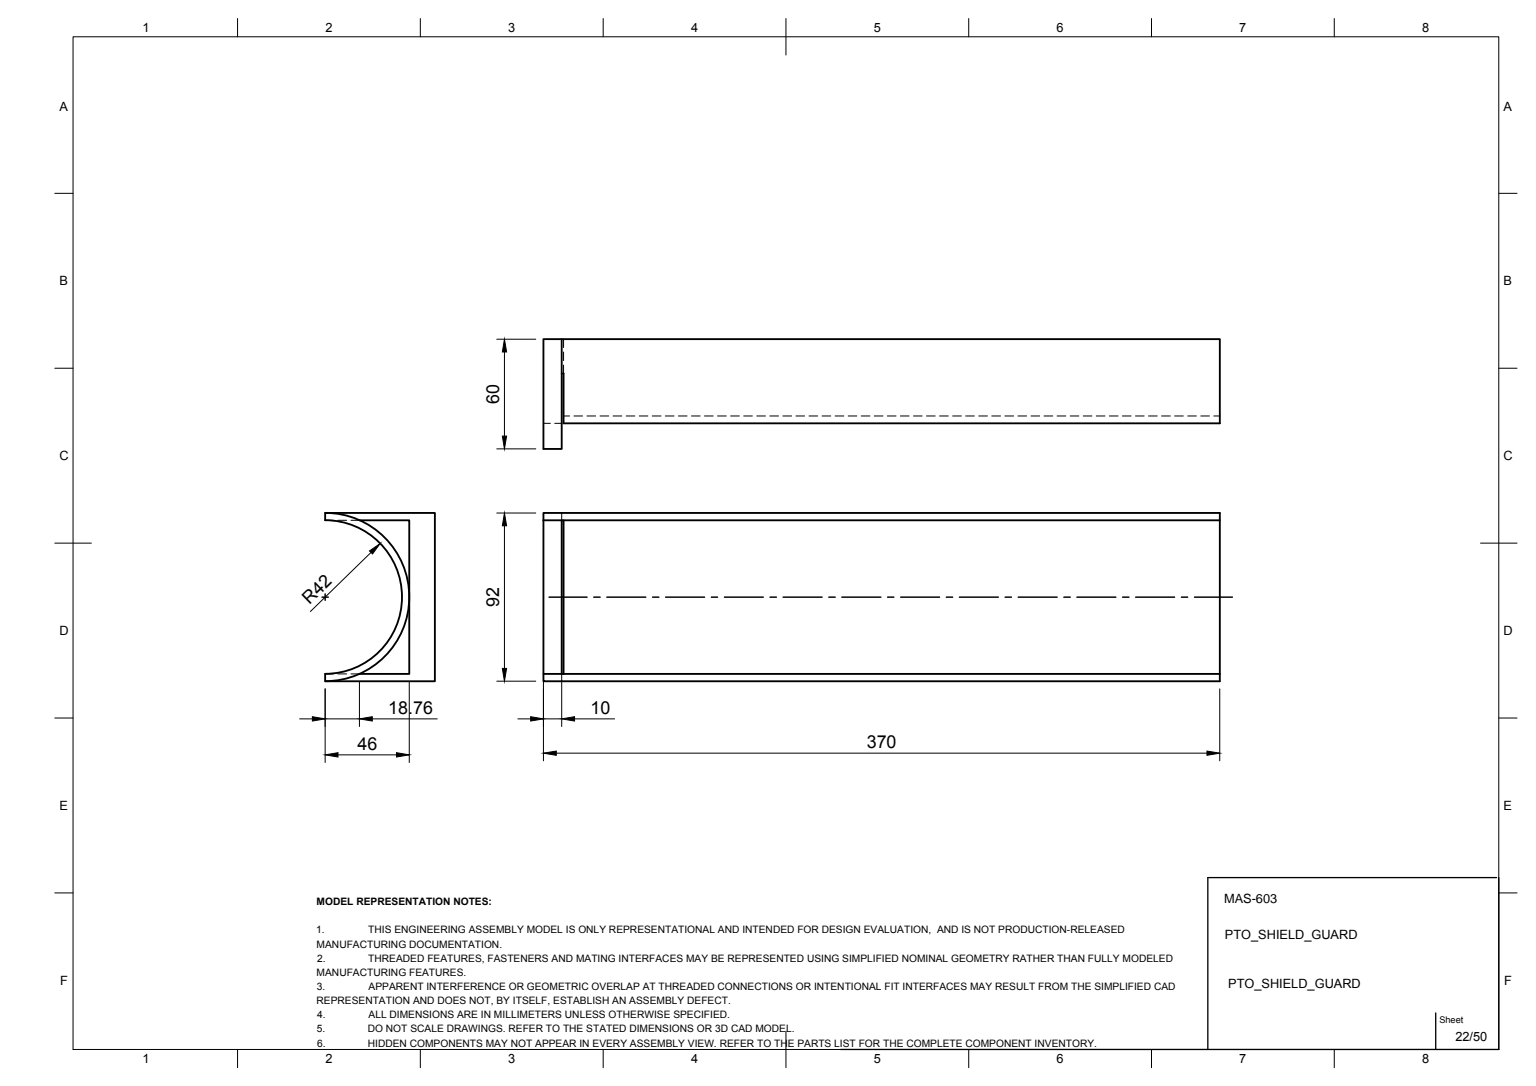
ISO-10303-21;
HEADER;
FILE_DESCRIPTION((''),'2;1');
FILE_NAME('PTO_SHIELD_GUARD.step','2026-10-01T22:06:14-07:00',(''),(''),'','','');
FILE_SCHEMA (('AUTOMOTIVE_DESIGN { 1 0 10303 214 3 1 1 }'));
ENDSEC;
DATA;
#10=MECHANICAL_DESIGN_GEOMETRIC_PRESENTATION_REPRESENTATION('',(#994),#50440);
#904=SHAPE_REPRESENTATION_RELATIONSHIP('SRR','None',#50636,#949) ;
#949=ADVANCED_BREP_SHAPE_REPRESENTATION('',(#1049),#50405) ;
#994=STYLED_ITEM('',(#50884),#1049) ;
#1049=MANIFOLD_SOLID_BREP('PTO_SHIELD_GUARD',#28661) ;
#2034=PLANE('',#30519) ;
#2035=PLANE('',#30522) ;
#2036=PLANE('',#30523) ;
#2037=PLANE('',#30524) ;
#2038=PLANE('',#30531) ;
#2039=PLANE('',#30532) ;
#2040=PLANE('',#30533) ;
#2041=PLANE('',#30534) ;
#2042=PLANE('',#30535) ;
#2043=PLANE('',#30536) ;
#2044=PLANE('',#30537) ;
#2045=PLANE('',#30538) ;
#3164=FACE_OUTER_BOUND('',#4905,.T.) ;
#3165=FACE_OUTER_BOUND('',#4906,.T.) ;
#3166=FACE_OUTER_BOUND('',#4907,.T.) ;
#3167=FACE_OUTER_BOUND('',#4908,.T.) ;
#3168=FACE_OUTER_BOUND('',#4909,.T.) ;
#3169=FACE_OUTER_BOUND('',#4910,.T.) ;
#3170=FACE_OUTER_BOUND('',#4911,.T.) ;
#3171=FACE_OUTER_BOUND('',#4912,.T.) ;
#3172=FACE_OUTER_BOUND('',#4913,.T.) ;
#3173=FACE_OUTER_BOUND('',#4914,.T.) ;
#3174=FACE_OUTER_BOUND('',#4915,.T.) ;
#3175=FACE_OUTER_BOUND('',#4916,.T.) ;
#3176=FACE_OUTER_BOUND('',#4917,.T.) ;
#3177=FACE_OUTER_BOUND('',#4918,.T.) ;
#4905=EDGE_LOOP('',(#22873,#22874,#22875,#22876)) ;
#4906=EDGE_LOOP('',(#22877,#22878,#22879,#22880,#22881,#22882)) ;
#4907=EDGE_LOOP('',(#22883,#22884,#22885,#22886)) ;
#4908=EDGE_LOOP('',(#22887,#22888,#22889,#22890,#22891,#22892)) ;
#4909=EDGE_LOOP('',(#22893,#22894,#22895,#22896,#22897,#22898,#22899,#22900)) ;
#4910=EDGE_LOOP('',(#22901,#22902,#22903,#22904)) ;
#4911=EDGE_LOOP('',(#22905,#22906,#22907,#22908,#22909,#22910)) ;
#4912=EDGE_LOOP('',(#22911,#22912,#22913,#22914,#22915,#22916,#22917,#22918)) ;
#4913=EDGE_LOOP('',(#22919,#22920,#22921,#22922,#22923,#22924,#22925,#22926)) ;
#4914=EDGE_LOOP('',(#22927,#22928,#22929,#22930)) ;
#4915=EDGE_LOOP('',(#22931,#22932,#22933,#22934)) ;
#4916=EDGE_LOOP('',(#22935,#22936,#22937,#22938)) ;
#4917=EDGE_LOOP('',(#22939,#22940,#22941,#22942,#22943,#22944)) ;
#4918=EDGE_LOOP('',(#22945,#22946,#22947,#22948)) ;
#7409=LINE('',#45813,#9881) ;
#7410=LINE('',#45816,#9882) ;
#7411=LINE('',#45819,#9883) ;
#7412=LINE('',#45821,#9884) ;
#7413=LINE('',#45823,#9885) ;
#7414=LINE('',#45825,#9886) ;
#7415=LINE('',#45826,#9887) ;
#7416=LINE('',#45829,#9888) ;
#7417=LINE('',#45831,#9889) ;
#7418=LINE('',#45832,#9890) ;
#7419=LINE('',#45835,#9891) ;
#7420=LINE('',#45836,#9892) ;
#7421=LINE('',#45838,#9893) ;
#7422=LINE('',#45839,#9894) ;
#7423=LINE('',#45844,#9895) ;
#7424=LINE('',#45848,#9896) ;
#7425=LINE('',#45852,#9897) ;
#7426=LINE('',#45855,#9898) ;
#7427=LINE('',#45858,#9899) ;
#7428=LINE('',#45859,#9900) ;
#7429=LINE('',#45860,#9901) ;
#7430=LINE('',#45863,#9902) ;
#7431=LINE('',#45865,#9903) ;
#7432=LINE('',#45867,#9904) ;
#7433=LINE('',#45868,#9905) ;
#7434=LINE('',#45871,#9906) ;
#7435=LINE('',#45873,#9907) ;
#7436=LINE('',#45874,#9908) ;
#7437=LINE('',#45876,#9909) ;
#7438=LINE('',#45877,#9910) ;
#7439=LINE('',#45880,#9911) ;
#7440=LINE('',#45882,#9912) ;
#9881=VECTOR('',#36676,1.) ;
#9882=VECTOR('',#36679,1.) ;
#9883=VECTOR('',#36682,1.) ;
#9884=VECTOR('',#36683,1.) ;
#9885=VECTOR('',#36684,1.) ;
#9886=VECTOR('',#36685,1.) ;
#9887=VECTOR('',#36686,1.) ;
#9888=VECTOR('',#36689,1.) ;
#9889=VECTOR('',#36690,1.) ;
#9890=VECTOR('',#36691,1.) ;
#9891=VECTOR('',#36694,1.) ;
#9892=VECTOR('',#36695,1.) ;
#9893=VECTOR('',#36696,1.) ;
#9894=VECTOR('',#36697,1.) ;
#9895=VECTOR('',#36702,1.) ;
#9896=VECTOR('',#36705,1.) ;
#9897=VECTOR('',#36710,1.) ;
#9898=VECTOR('',#36713,1.) ;
#9899=VECTOR('',#36716,1.) ;
#9900=VECTOR('',#36717,1.) ;
#9901=VECTOR('',#36718,1.) ;
#9902=VECTOR('',#36721,1.) ;
#9903=VECTOR('',#36722,1.) ;
#9904=VECTOR('',#36723,1.) ;
#9905=VECTOR('',#36724,1.) ;
#9906=VECTOR('',#36727,1.) ;
#9907=VECTOR('',#36728,1.) ;
#9908=VECTOR('',#36729,1.) ;
#9909=VECTOR('',#36732,1.) ;
#9910=VECTOR('',#36733,1.) ;
#9911=VECTOR('',#36738,1.) ;
#9912=VECTOR('',#36741,1.) ;
#11097=CIRCLE('',#30520,4.6) ;
#11098=CIRCLE('',#30521,4.2) ;
#11099=CIRCLE('',#30526,4.6) ;
#11100=CIRCLE('',#30527,4.6) ;
#11101=CIRCLE('',#30528,4.6) ;
#11102=CIRCLE('',#30530,4.2) ;
#13275=VERTEX_POINT('',#45809) ;
#13276=VERTEX_POINT('',#45810) ;
#13277=VERTEX_POINT('',#45812) ;
#13278=VERTEX_POINT('',#45814) ;
#13279=VERTEX_POINT('',#45818) ;
#13280=VERTEX_POINT('',#45820) ;
#13281=VERTEX_POINT('',#45822) ;
#13282=VERTEX_POINT('',#45824) ;
#13283=VERTEX_POINT('',#45828) ;
#13284=VERTEX_POINT('',#45830) ;
#13285=VERTEX_POINT('',#45834) ;
#13286=VERTEX_POINT('',#45837) ;
#13287=VERTEX_POINT('',#45841) ;
#13288=VERTEX_POINT('',#45843) ;
#13289=VERTEX_POINT('',#45845) ;
#13290=VERTEX_POINT('',#45847) ;
#13291=VERTEX_POINT('',#45851) ;
#13292=VERTEX_POINT('',#45853) ;
#13293=VERTEX_POINT('',#45857) ;
#13294=VERTEX_POINT('',#45862) ;
#13295=VERTEX_POINT('',#45864) ;
#13296=VERTEX_POINT('',#45866) ;
#13297=VERTEX_POINT('',#45870) ;
#13298=VERTEX_POINT('',#45872) ;
#16702=EDGE_CURVE('',#13275,#13276,#11097,.T.) ;
#16703=EDGE_CURVE('',#13275,#13277,#7409,.T.) ;
#16704=EDGE_CURVE('',#13278,#13277,#11098,.T.) ;
#16705=EDGE_CURVE('',#13276,#13278,#7410,.T.) ;
#16706=EDGE_CURVE('',#13276,#13279,#7411,.T.) ;
#16707=EDGE_CURVE('',#13278,#13280,#7412,.T.) ;
#16708=EDGE_CURVE('',#13281,#13280,#7413,.T.) ;
#16709=EDGE_CURVE('',#13281,#13282,#7414,.T.) ;
#16710=EDGE_CURVE('',#13279,#13282,#7415,.T.) ;
#16711=EDGE_CURVE('',#13282,#13283,#7416,.T.) ;
#16712=EDGE_CURVE('',#13284,#13281,#7417,.T.) ;
#16713=EDGE_CURVE('',#13283,#13284,#7418,.T.) ;
#16714=EDGE_CURVE('',#13285,#13275,#7419,.T.) ;
#16715=EDGE_CURVE('',#13283,#13285,#7420,.T.) ;
#16716=EDGE_CURVE('',#13286,#13284,#7421,.T.) ;
#16717=EDGE_CURVE('',#13286,#13277,#7422,.T.) ;
#16718=EDGE_CURVE('',#13279,#13287,#11099,.T.) ;
#16719=EDGE_CURVE('',#13287,#13288,#7423,.T.) ;
#16720=EDGE_CURVE('',#13289,#13288,#11100,.T.) ;
#16721=EDGE_CURVE('',#13289,#13290,#7424,.T.) ;
#16722=EDGE_CURVE('',#13290,#13285,#11101,.T.) ;
#16723=EDGE_CURVE('',#13277,#13291,#7425,.T.) ;
#16724=EDGE_CURVE('',#13292,#13291,#11102,.T.) ;
#16725=EDGE_CURVE('',#13292,#13278,#7426,.T.) ;
#16726=EDGE_CURVE('',#13293,#13286,#7427,.T.) ;
#16727=EDGE_CURVE('',#13290,#13293,#7428,.T.) ;
#16728=EDGE_CURVE('',#13291,#13289,#7429,.T.) ;
#16729=EDGE_CURVE('',#13280,#13294,#7430,.T.) ;
#16730=EDGE_CURVE('',#13295,#13294,#7431,.T.) ;
#16731=EDGE_CURVE('',#13296,#13295,#7432,.T.) ;
#16732=EDGE_CURVE('',#13296,#13293,#7433,.T.) ;
#16733=EDGE_CURVE('',#13297,#13290,#7434,.T.) ;
#16734=EDGE_CURVE('',#13298,#13297,#7435,.T.) ;
#16735=EDGE_CURVE('',#13298,#13287,#7436,.T.) ;
#16736=EDGE_CURVE('',#13295,#13298,#7437,.T.) ;
#16737=EDGE_CURVE('',#13297,#13296,#7438,.T.) ;
#16738=EDGE_CURVE('',#13294,#13287,#7439,.T.) ;
#16739=EDGE_CURVE('',#13288,#13292,#7440,.T.) ;
#22873=ORIENTED_EDGE('',*,*,#16702,.F.) ;
#22874=ORIENTED_EDGE('',*,*,#16703,.T.) ;
#22875=ORIENTED_EDGE('',*,*,#16704,.F.) ;
#22876=ORIENTED_EDGE('',*,*,#16705,.F.) ;
#22877=ORIENTED_EDGE('',*,*,#16706,.F.) ;
#22878=ORIENTED_EDGE('',*,*,#16705,.T.) ;
#22879=ORIENTED_EDGE('',*,*,#16707,.T.) ;
#22880=ORIENTED_EDGE('',*,*,#16708,.F.) ;
#22881=ORIENTED_EDGE('',*,*,#16709,.T.) ;
#22882=ORIENTED_EDGE('',*,*,#16710,.F.) ;
#22883=ORIENTED_EDGE('',*,*,#16711,.F.) ;
#22884=ORIENTED_EDGE('',*,*,#16709,.F.) ;
#22885=ORIENTED_EDGE('',*,*,#16712,.F.) ;
#22886=ORIENTED_EDGE('',*,*,#16713,.F.) ;
#22887=ORIENTED_EDGE('',*,*,#16714,.F.) ;
#22888=ORIENTED_EDGE('',*,*,#16715,.F.) ;
#22889=ORIENTED_EDGE('',*,*,#16713,.T.) ;
#22890=ORIENTED_EDGE('',*,*,#16716,.F.) ;
#22891=ORIENTED_EDGE('',*,*,#16717,.T.) ;
#22892=ORIENTED_EDGE('',*,*,#16703,.F.) ;
#22893=ORIENTED_EDGE('',*,*,#16714,.T.) ;
#22894=ORIENTED_EDGE('',*,*,#16702,.T.) ;
#22895=ORIENTED_EDGE('',*,*,#16706,.T.) ;
#22896=ORIENTED_EDGE('',*,*,#16718,.T.) ;
#22897=ORIENTED_EDGE('',*,*,#16719,.T.) ;
#22898=ORIENTED_EDGE('',*,*,#16720,.F.) ;
#22899=ORIENTED_EDGE('',*,*,#16721,.T.) ;
#22900=ORIENTED_EDGE('',*,*,#16722,.T.) ;
#22901=ORIENTED_EDGE('',*,*,#16704,.T.) ;
#22902=ORIENTED_EDGE('',*,*,#16723,.T.) ;
#22903=ORIENTED_EDGE('',*,*,#16724,.F.) ;
#22904=ORIENTED_EDGE('',*,*,#16725,.T.) ;
#22905=ORIENTED_EDGE('',*,*,#16717,.F.) ;
#22906=ORIENTED_EDGE('',*,*,#16726,.F.) ;
#22907=ORIENTED_EDGE('',*,*,#16727,.F.) ;
#22908=ORIENTED_EDGE('',*,*,#16721,.F.) ;
#22909=ORIENTED_EDGE('',*,*,#16728,.F.) ;
#22910=ORIENTED_EDGE('',*,*,#16723,.F.) ;
#22911=ORIENTED_EDGE('',*,*,#16716,.T.) ;
#22912=ORIENTED_EDGE('',*,*,#16712,.T.) ;
#22913=ORIENTED_EDGE('',*,*,#16708,.T.) ;
#22914=ORIENTED_EDGE('',*,*,#16729,.T.) ;
#22915=ORIENTED_EDGE('',*,*,#16730,.F.) ;
#22916=ORIENTED_EDGE('',*,*,#16731,.F.) ;
#22917=ORIENTED_EDGE('',*,*,#16732,.T.) ;
#22918=ORIENTED_EDGE('',*,*,#16726,.T.) ;
#22919=ORIENTED_EDGE('',*,*,#16715,.T.) ;
#22920=ORIENTED_EDGE('',*,*,#16722,.F.) ;
#22921=ORIENTED_EDGE('',*,*,#16733,.F.) ;
#22922=ORIENTED_EDGE('',*,*,#16734,.F.) ;
#22923=ORIENTED_EDGE('',*,*,#16735,.T.) ;
#22924=ORIENTED_EDGE('',*,*,#16718,.F.) ;
#22925=ORIENTED_EDGE('',*,*,#16710,.T.) ;
#22926=ORIENTED_EDGE('',*,*,#16711,.T.) ;
#22927=ORIENTED_EDGE('',*,*,#16731,.T.) ;
#22928=ORIENTED_EDGE('',*,*,#16736,.T.) ;
#22929=ORIENTED_EDGE('',*,*,#16734,.T.) ;
#22930=ORIENTED_EDGE('',*,*,#16737,.T.) ;
#22931=ORIENTED_EDGE('',*,*,#16733,.T.) ;
#22932=ORIENTED_EDGE('',*,*,#16727,.T.) ;
#22933=ORIENTED_EDGE('',*,*,#16732,.F.) ;
#22934=ORIENTED_EDGE('',*,*,#16737,.F.) ;
#22935=ORIENTED_EDGE('',*,*,#16730,.T.) ;
#22936=ORIENTED_EDGE('',*,*,#16738,.T.) ;
#22937=ORIENTED_EDGE('',*,*,#16735,.F.) ;
#22938=ORIENTED_EDGE('',*,*,#16736,.F.) ;
#22939=ORIENTED_EDGE('',*,*,#16707,.F.) ;
#22940=ORIENTED_EDGE('',*,*,#16725,.F.) ;
#22941=ORIENTED_EDGE('',*,*,#16739,.F.) ;
#22942=ORIENTED_EDGE('',*,*,#16719,.F.) ;
#22943=ORIENTED_EDGE('',*,*,#16738,.F.) ;
#22944=ORIENTED_EDGE('',*,*,#16729,.F.) ;
#22945=ORIENTED_EDGE('',*,*,#16739,.T.) ;
#22946=ORIENTED_EDGE('',*,*,#16724,.T.) ;
#22947=ORIENTED_EDGE('',*,*,#16728,.T.) ;
#22948=ORIENTED_EDGE('',*,*,#16720,.T.) ;
#26819=CYLINDRICAL_SURFACE('',#30525,4.6) ;
#26820=CYLINDRICAL_SURFACE('',#30529,4.2) ;
#27899=ADVANCED_FACE('',(#3164),#2034,.T.) ;
#27900=ADVANCED_FACE('',(#3165),#2035,.T.) ;
#27901=ADVANCED_FACE('',(#3166),#2036,.F.) ;
#27902=ADVANCED_FACE('',(#3167),#2037,.T.) ;
#27903=ADVANCED_FACE('',(#3168),#26819,.T.) ;
#27904=ADVANCED_FACE('',(#3169),#26820,.F.) ;
#27905=ADVANCED_FACE('',(#3170),#2038,.F.) ;
#27906=ADVANCED_FACE('',(#3171),#2039,.T.) ;
#27907=ADVANCED_FACE('',(#3172),#2040,.F.) ;
#27908=ADVANCED_FACE('',(#3173),#2041,.T.) ;
#27909=ADVANCED_FACE('',(#3174),#2042,.F.) ;
#27910=ADVANCED_FACE('',(#3175),#2043,.F.) ;
#27911=ADVANCED_FACE('',(#3176),#2044,.F.) ;
#27912=ADVANCED_FACE('',(#3177),#2045,.T.) ;
#28661=CLOSED_SHELL('',(#27899,#27900,#27901,#27902,#27903,#27904,#27905,
#27906,#27907,#27908,#27909,#27910,#27911,#27912)) ;
#30518=AXIS2_PLACEMENT_3D('',#45807,#36670,#36671) ;
#30519=AXIS2_PLACEMENT_3D('',#45808,#36672,#36673) ;
#30520=AXIS2_PLACEMENT_3D('',#45811,#36674,#36675) ;
#30521=AXIS2_PLACEMENT_3D('',#45815,#36677,#36678) ;
#30522=AXIS2_PLACEMENT_3D('',#45817,#36680,#36681) ;
#30523=AXIS2_PLACEMENT_3D('',#45827,#36687,#36688) ;
#30524=AXIS2_PLACEMENT_3D('',#45833,#36692,#36693) ;
#30525=AXIS2_PLACEMENT_3D('',#45840,#36698,#36699) ;
#30526=AXIS2_PLACEMENT_3D('',#45842,#36700,#36701) ;
#30527=AXIS2_PLACEMENT_3D('',#45846,#36703,#36704) ;
#30528=AXIS2_PLACEMENT_3D('',#45849,#36706,#36707) ;
#30529=AXIS2_PLACEMENT_3D('',#45850,#36708,#36709) ;
#30530=AXIS2_PLACEMENT_3D('',#45854,#36711,#36712) ;
#30531=AXIS2_PLACEMENT_3D('',#45856,#36714,#36715) ;
#30532=AXIS2_PLACEMENT_3D('',#45861,#36719,#36720) ;
#30533=AXIS2_PLACEMENT_3D('',#45869,#36725,#36726) ;
#30534=AXIS2_PLACEMENT_3D('',#45875,#36730,#36731) ;
#30535=AXIS2_PLACEMENT_3D('',#45878,#36734,#36735) ;
#30536=AXIS2_PLACEMENT_3D('',#45879,#36736,#36737) ;
#30537=AXIS2_PLACEMENT_3D('',#45881,#36739,#36740) ;
#30538=AXIS2_PLACEMENT_3D('',#45883,#36742,#36743) ;
#36670=DIRECTION('axis',(0.,0.,1.)) ;
#36671=DIRECTION('refdir',(1.,0.,0.)) ;
#36672=DIRECTION('center_axis',(1.,0.,0.)) ;
#36673=DIRECTION('ref_axis',(0.,0.,-1.)) ;
#36674=DIRECTION('center_axis',(-1.,0.,0.)) ;
#36675=DIRECTION('ref_axis',(0.,0.,-1.)) ;
#36676=DIRECTION('',(0.,0.,-1.)) ;
#36677=DIRECTION('center_axis',(1.,0.,0.)) ;
#36678=DIRECTION('ref_axis',(0.,0.,-1.)) ;
#36679=DIRECTION('',(0.,0.,-1.)) ;
#36680=DIRECTION('center_axis',(0.,-1.,0.)) ;
#36681=DIRECTION('ref_axis',(0.,0.,-1.)) ;
#36682=DIRECTION('',(1.,0.,0.)) ;
#36683=DIRECTION('',(1.,0.,0.)) ;
#36684=DIRECTION('',(0.,0.,-1.)) ;
#36685=DIRECTION('',(-1.,0.,0.)) ;
#36686=DIRECTION('',(0.,0.,1.)) ;
#36687=DIRECTION('center_axis',(0.,0.,1.)) ;
#36688=DIRECTION('ref_axis',(1.,0.,0.)) ;
#36689=DIRECTION('',(0.,-1.,0.)) ;
#36690=DIRECTION('',(0.,1.,0.)) ;
#36691=DIRECTION('',(1.,0.,0.)) ;
#36692=DIRECTION('center_axis',(0.,1.,0.)) ;
#36693=DIRECTION('ref_axis',(0.,0.,1.)) ;
#36694=DIRECTION('',(-1.,0.,0.)) ;
#36695=DIRECTION('',(0.,0.,-1.)) ;
#36696=DIRECTION('',(0.,0.,1.)) ;
#36697=DIRECTION('',(-1.,0.,0.)) ;
#36698=DIRECTION('center_axis',(1.,0.,0.)) ;
#36699=DIRECTION('ref_axis',(0.,-1.22464679914735E-16,1.)) ;
#36700=DIRECTION('center_axis',(-1.,0.,0.)) ;
#36701=DIRECTION('ref_axis',(0.,0.,-1.)) ;
#36702=DIRECTION('',(-1.,0.,0.)) ;
#36703=DIRECTION('center_axis',(-1.,0.,0.)) ;
#36704=DIRECTION('ref_axis',(0.,0.,-1.)) ;
#36705=DIRECTION('',(1.,0.,0.)) ;
#36706=DIRECTION('center_axis',(-1.,0.,0.)) ;
#36707=DIRECTION('ref_axis',(0.,0.,-1.)) ;
#36708=DIRECTION('center_axis',(1.,0.,0.)) ;
#36709=DIRECTION('ref_axis',(0.,1.22464679914735E-16,1.)) ;
#36710=DIRECTION('',(-1.,0.,0.)) ;
#36711=DIRECTION('center_axis',(1.,0.,0.)) ;
#36712=DIRECTION('ref_axis',(0.,0.,-1.)) ;
#36713=DIRECTION('',(1.,0.,0.)) ;
#36714=DIRECTION('center_axis',(0.,0.,1.)) ;
#36715=DIRECTION('ref_axis',(1.,0.,0.)) ;
#36716=DIRECTION('',(0.,1.,0.)) ;
#36717=DIRECTION('',(1.,0.,0.)) ;
#36718=DIRECTION('',(0.,-1.,0.)) ;
#36719=DIRECTION('center_axis',(1.,0.,0.)) ;
#36720=DIRECTION('ref_axis',(0.,0.,-1.)) ;
#36721=DIRECTION('',(0.,1.,0.)) ;
#36722=DIRECTION('',(0.,0.,-1.)) ;
#36723=DIRECTION('',(0.,1.,0.)) ;
#36724=DIRECTION('',(0.,0.,-1.)) ;
#36725=DIRECTION('center_axis',(1.,0.,0.)) ;
#36726=DIRECTION('ref_axis',(0.,0.,-1.)) ;
#36727=DIRECTION('',(0.,0.,-1.)) ;
#36728=DIRECTION('',(0.,-1.,0.)) ;
#36729=DIRECTION('',(0.,0.,-1.)) ;
#36730=DIRECTION('center_axis',(0.,0.,1.)) ;
#36731=DIRECTION('ref_axis',(1.,0.,0.)) ;
#36732=DIRECTION('',(-1.,0.,0.)) ;
#36733=DIRECTION('',(1.,0.,0.)) ;
#36734=DIRECTION('center_axis',(0.,1.,0.)) ;
#36735=DIRECTION('ref_axis',(0.,0.,1.)) ;
#36736=DIRECTION('center_axis',(0.,-1.,0.)) ;
#36737=DIRECTION('ref_axis',(0.,0.,-1.)) ;
#36738=DIRECTION('',(-1.,0.,0.)) ;
#36739=DIRECTION('center_axis',(0.,0.,1.)) ;
#36740=DIRECTION('ref_axis',(1.,0.,0.)) ;
#36741=DIRECTION('',(0.,-1.,0.)) ;
#36742=DIRECTION('center_axis',(-1.,0.,0.)) ;
#36743=DIRECTION('ref_axis',(0.,0.,1.)) ;
#45807=CARTESIAN_POINT('',(0.,0.,0.)) ;
#45808=CARTESIAN_POINT('Origin',(-16.1,0.,36.3)) ;
#45809=CARTESIAN_POINT('',(-16.1,-4.2,35.8761663039294)) ;
#45810=CARTESIAN_POINT('',(-16.1,4.2,35.8761663039294)) ;
#45811=CARTESIAN_POINT('Origin',(-16.1,0.,34.)) ;
#45812=CARTESIAN_POINT('',(-16.1,-4.2,34.)) ;
#45813=CARTESIAN_POINT('',(-16.1,-4.2,36.3)) ;
#45814=CARTESIAN_POINT('',(-16.1,4.2,34.)) ;
#45815=CARTESIAN_POINT('Origin',(-16.1,0.,34.)) ;
#45816=CARTESIAN_POINT('',(-16.1,4.2,36.3)) ;
#45817=CARTESIAN_POINT('Origin',(-15.5,4.2,36.3)) ;
#45818=CARTESIAN_POINT('',(-16.,4.2,35.8761663039294)) ;
#45819=CARTESIAN_POINT('',(-33.5,4.2,35.8761663039294)) ;
#45820=CARTESIAN_POINT('',(-15.,4.2,34.)) ;
#45821=CARTESIAN_POINT('',(-33.5,4.2,34.)) ;
#45822=CARTESIAN_POINT('',(-15.,4.2,38.6)) ;
#45823=CARTESIAN_POINT('',(-15.,4.2,35.15)) ;
#45824=CARTESIAN_POINT('',(-16.,4.2,38.6)) ;
#45825=CARTESIAN_POINT('',(-15.5,4.2,38.6)) ;
#45826=CARTESIAN_POINT('',(-16.,4.2,36.65)) ;
#45827=CARTESIAN_POINT('Origin',(-15.5,0.,38.6)) ;
#45828=CARTESIAN_POINT('',(-16.,-4.2,38.6)) ;
#45829=CARTESIAN_POINT('',(-16.,0.,38.6)) ;
#45830=CARTESIAN_POINT('',(-15.,-4.2,38.6)) ;
#45831=CARTESIAN_POINT('',(-15.,0.,38.6)) ;
#45832=CARTESIAN_POINT('',(-15.5,-4.2,38.6)) ;
#45833=CARTESIAN_POINT('Origin',(-15.5,-4.2,36.3)) ;
#45834=CARTESIAN_POINT('',(-16.,-4.2,35.8761663039294)) ;
#45835=CARTESIAN_POINT('',(-33.5,-4.2,35.8761663039294)) ;
#45836=CARTESIAN_POINT('',(-16.,-4.2,36.65)) ;
#45837=CARTESIAN_POINT('',(-15.,-4.2,34.)) ;
#45838=CARTESIAN_POINT('',(-15.,-4.2,35.15)) ;
#45839=CARTESIAN_POINT('',(-33.5,-4.2,34.)) ;
#45840=CARTESIAN_POINT('Origin',(-33.5,0.,34.)) ;
#45841=CARTESIAN_POINT('',(-16.,4.6,34.)) ;
#45842=CARTESIAN_POINT('Origin',(-16.,0.,34.)) ;
#45843=CARTESIAN_POINT('',(-52.,4.6,34.)) ;
#45844=CARTESIAN_POINT('',(-33.5,4.6,34.)) ;
#45845=CARTESIAN_POINT('',(-52.,-4.6,34.)) ;
#45846=CARTESIAN_POINT('Origin',(-52.,0.,34.)) ;
#45847=CARTESIAN_POINT('',(-16.,-4.6,34.)) ;
#45848=CARTESIAN_POINT('',(-33.5,-4.6,34.)) ;
#45849=CARTESIAN_POINT('Origin',(-16.,0.,34.)) ;
#45850=CARTESIAN_POINT('Origin',(-33.5,0.,34.)) ;
#45851=CARTESIAN_POINT('',(-52.,-4.2,34.)) ;
#45852=CARTESIAN_POINT('',(-33.5,-4.2,34.)) ;
#45853=CARTESIAN_POINT('',(-52.,4.2,34.)) ;
#45854=CARTESIAN_POINT('Origin',(-52.,0.,34.)) ;
#45855=CARTESIAN_POINT('',(-33.5,4.2,34.)) ;
#45856=CARTESIAN_POINT('Origin',(-33.5,0.,34.)) ;
#45857=CARTESIAN_POINT('',(-15.,-4.6,34.)) ;
#45858=CARTESIAN_POINT('',(-15.,0.,34.)) ;
#45859=CARTESIAN_POINT('',(-33.5,-4.6,34.)) ;
#45860=CARTESIAN_POINT('',(-52.,0.,34.)) ;
#45861=CARTESIAN_POINT('Origin',(-15.,0.,34.)) ;
#45862=CARTESIAN_POINT('',(-15.,4.6,34.)) ;
#45863=CARTESIAN_POINT('',(-15.,0.,34.)) ;
#45864=CARTESIAN_POINT('',(-15.,4.6,40.)) ;
#45865=CARTESIAN_POINT('',(-15.,4.6,37.)) ;
#45866=CARTESIAN_POINT('',(-15.,-4.6,40.)) ;
#45867=CARTESIAN_POINT('',(-15.,0.,40.)) ;
#45868=CARTESIAN_POINT('',(-15.,-4.6,37.)) ;
#45869=CARTESIAN_POINT('Origin',(-16.,0.,37.)) ;
#45870=CARTESIAN_POINT('',(-16.,-4.6,40.)) ;
#45871=CARTESIAN_POINT('',(-16.,-4.6,37.)) ;
#45872=CARTESIAN_POINT('',(-16.,4.6,40.)) ;
#45873=CARTESIAN_POINT('',(-16.,0.,40.)) ;
#45874=CARTESIAN_POINT('',(-16.,4.6,37.)) ;
#45875=CARTESIAN_POINT('Origin',(-15.5,0.,40.)) ;
#45876=CARTESIAN_POINT('',(-15.5,4.6,40.)) ;
#45877=CARTESIAN_POINT('',(-15.5,-4.6,40.)) ;
#45878=CARTESIAN_POINT('Origin',(-15.5,-4.6,37.)) ;
#45879=CARTESIAN_POINT('Origin',(-15.5,4.6,37.)) ;
#45880=CARTESIAN_POINT('',(-33.5,4.6,34.)) ;
#45881=CARTESIAN_POINT('Origin',(-33.5,0.,34.)) ;
#45882=CARTESIAN_POINT('',(-52.,0.,34.)) ;
#45883=CARTESIAN_POINT('Origin',(-52.,0.,34.)) ;
#50352=UNCERTAINTY_MEASURE_WITH_UNIT(LENGTH_MEASURE(0.001),#50441,
'DISTANCE_ACCURACY_VALUE',
'Maximum model space distance between geometric entities at asserted c
onnectivities') ;
#50387=UNCERTAINTY_MEASURE_WITH_UNIT(LENGTH_MEASURE(0.001),#50441,
'DISTANCE_ACCURACY_VALUE',
'Maximum model space distance between geometric entities at asserted c
onnectivities') ;
#50405=(
GEOMETRIC_REPRESENTATION_CONTEXT(3)
GLOBAL_UNCERTAINTY_ASSIGNED_CONTEXT((#50352))
GLOBAL_UNIT_ASSIGNED_CONTEXT((#50441,#50443,#50444))
REPRESENTATION_CONTEXT('','3D')
) ;
#50440=(
GEOMETRIC_REPRESENTATION_CONTEXT(3)
GLOBAL_UNCERTAINTY_ASSIGNED_CONTEXT((#50387))
GLOBAL_UNIT_ASSIGNED_CONTEXT((#50441,#50443,#50444))
REPRESENTATION_CONTEXT('','3D')
) ;
#50441=(
LENGTH_UNIT()
NAMED_UNIT(*)
SI_UNIT(.CENTI.,.METRE.)
) ;
#50443=(
NAMED_UNIT(*)
PLANE_ANGLE_UNIT()
SI_UNIT($,.RADIAN.)
) ;
#50444=(
NAMED_UNIT(*)
SI_UNIT($,.STERADIAN.)
SOLID_ANGLE_UNIT()
) ;
#50462=SHAPE_DEFINITION_REPRESENTATION(#50528,#50636) ;
#50528=PRODUCT_DEFINITION_SHAPE('',$,#50689) ;
#50636=SHAPE_REPRESENTATION('',(#30518),#50405) ;
#50671=PRODUCT_DEFINITION_CONTEXT('part definition',#50829,'design') ;
#50689=PRODUCT_DEFINITION('PTO_SHIELD_GUARD','PTO_SHIELD_GUARD',
#50741,#50671) ;
#50741=PRODUCT_DEFINITION_FORMATION('',$,#50848) ;
#50829=APPLICATION_CONTEXT(
'Core Data for Automotive Mechanical Design Process') ;
#50830=PRODUCT_CONTEXT('part definition',#50829,'mechanical') ;
#50848=PRODUCT('PTO_SHIELD_GUARD','PTO_SHIELD_GUARD',$,(#50830)) ;
#50884=PRESENTATION_STYLE_ASSIGNMENT((#50891)) ;
#50891=SURFACE_STYLE_USAGE(.BOTH.,#50898) ;
#50898=SURFACE_SIDE_STYLE('',(#50905)) ;
#50905=SURFACE_STYLE_FILL_AREA(#50912) ;
#50912=FILL_AREA_STYLE('Surface - Matte',(#50919)) ;
#50919=FILL_AREA_STYLE_COLOUR('Surface - Matte',#50926) ;
#50926=COLOUR_RGB('Surface - Matte', 0.72549020, 0.75294118, 0.79215686) ;
ENDSEC;
END-ISO-10303-21;
